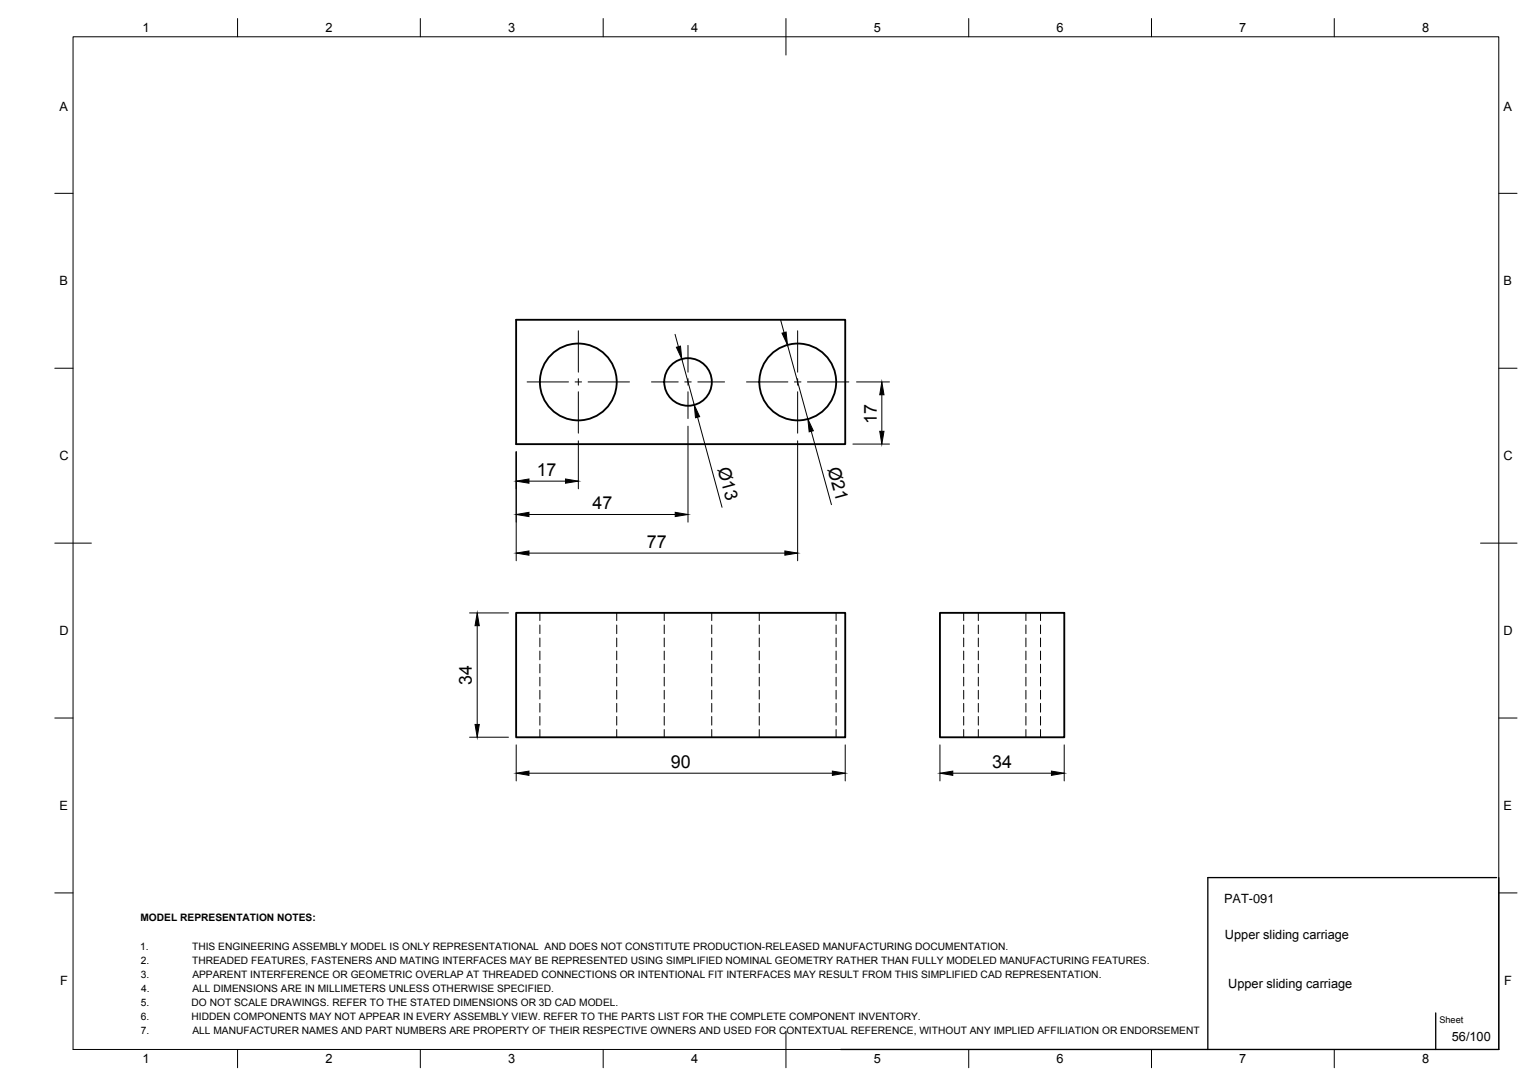
ISO-10303-21;
HEADER;
/* Generated by software containing ST-Developer
 * from STEP Tools, Inc. (www.steptools.com) 
 */

FILE_DESCRIPTION(
/* description */ ('PAT-091'),
/* implementation_level */ '2;1');

FILE_NAME(
/* name */ 'Upper sliding carriage.step',
/* time_stamp */ '2026-10-27T15:34:44-07:00',
/* author */ (''),
/* organization */ (''),
/* preprocessor_version */ 'ST-DEVELOPER v20.2',
/* originating_system */ 'Autodesk Translation Framework v15.17.0.0',
/* authorisation */ '');

FILE_SCHEMA (('AUTOMOTIVE_DESIGN { 1 0 10303 214 3 1 1 }'));
ENDSEC;

DATA;
#10=MECHANICAL_DESIGN_GEOMETRIC_PRESENTATION_REPRESENTATION('',(#1013),#25100);
#793=SHAPE_REPRESENTATION_RELATIONSHIP('SRR','None',#25557,#903);
#903=ADVANCED_BREP_SHAPE_REPRESENTATION('',(#1135),#25027);
#1013=STYLED_ITEM('',(#26177),#1135);
#1135=MANIFOLD_SOLID_BREP('Body1',#13292);
#1432=FACE_BOUND('',#3439,.T.);
#1433=FACE_BOUND('',#3440,.T.);
#1434=FACE_BOUND('',#3441,.T.);
#1435=FACE_BOUND('',#3444,.T.);
#1436=FACE_BOUND('',#3445,.T.);
#1437=FACE_BOUND('',#3446,.T.);
#1823=PLANE('',#15279);
#1824=PLANE('',#15280);
#1825=PLANE('',#15281);
#1826=PLANE('',#15282);
#1827=PLANE('',#15283);
#1828=PLANE('',#15284);
#2399=FACE_OUTER_BOUND('',#3434,.T.);
#2400=FACE_OUTER_BOUND('',#3435,.T.);
#2401=FACE_OUTER_BOUND('',#3436,.T.);
#2402=FACE_OUTER_BOUND('',#3437,.T.);
#2403=FACE_OUTER_BOUND('',#3438,.T.);
#2404=FACE_OUTER_BOUND('',#3442,.T.);
#2405=FACE_OUTER_BOUND('',#3443,.T.);
#2406=FACE_OUTER_BOUND('',#3447,.T.);
#2407=FACE_OUTER_BOUND('',#3448,.T.);
#3434=EDGE_LOOP('',(#10344,#10345,#10346,#10347));
#3435=EDGE_LOOP('',(#10348,#10349,#10350,#10351));
#3436=EDGE_LOOP('',(#10352,#10353,#10354,#10355));
#3437=EDGE_LOOP('',(#10356,#10357,#10358,#10359));
#3438=EDGE_LOOP('',(#10360,#10361,#10362,#10363));
#3439=EDGE_LOOP('',(#10364));
#3440=EDGE_LOOP('',(#10365));
#3441=EDGE_LOOP('',(#10366));
#3442=EDGE_LOOP('',(#10367,#10368,#10369,#10370));
#3443=EDGE_LOOP('',(#10371,#10372,#10373,#10374));
#3444=EDGE_LOOP('',(#10375));
#3445=EDGE_LOOP('',(#10376));
#3446=EDGE_LOOP('',(#10377));
#3447=EDGE_LOOP('',(#10378,#10379,#10380,#10381));
#3448=EDGE_LOOP('',(#10382,#10383,#10384,#10385));
#4507=LINE('',#22529,#5247);
#4508=LINE('',#22535,#5248);
#4509=LINE('',#22541,#5249);
#4510=LINE('',#22546,#5250);
#4511=LINE('',#22548,#5251);
#4512=LINE('',#22550,#5252);
#4513=LINE('',#22551,#5253);
#4514=LINE('',#22554,#5254);
#4515=LINE('',#22556,#5255);
#4516=LINE('',#22557,#5256);
#4517=LINE('',#22560,#5257);
#4518=LINE('',#22562,#5258);
#4519=LINE('',#22563,#5259);
#4520=LINE('',#22565,#5260);
#4521=LINE('',#22566,#5261);
#5247=VECTOR('',#18225,0.65);
#5248=VECTOR('',#18232,1.05);
#5249=VECTOR('',#18239,1.05);
#5250=VECTOR('',#18244,1.);
#5251=VECTOR('',#18245,1.);
#5252=VECTOR('',#18246,1.);
#5253=VECTOR('',#18247,1.);
#5254=VECTOR('',#18250,1.);
#5255=VECTOR('',#18251,1.);
#5256=VECTOR('',#18252,1.);
#5257=VECTOR('',#18255,1.);
#5258=VECTOR('',#18256,1.);
#5259=VECTOR('',#18257,1.);
#5260=VECTOR('',#18260,1.);
#5261=VECTOR('',#18261,1.);
#5905=CIRCLE('',#15271,0.65);
#5906=CIRCLE('',#15272,0.65);
#5907=CIRCLE('',#15274,1.05);
#5908=CIRCLE('',#15275,1.05);
#5909=CIRCLE('',#15277,1.05);
#5910=CIRCLE('',#15278,1.05);
#6838=VERTEX_POINT('',#22526);
#6839=VERTEX_POINT('',#22528);
#6840=VERTEX_POINT('',#22532);
#6841=VERTEX_POINT('',#22534);
#6842=VERTEX_POINT('',#22538);
#6843=VERTEX_POINT('',#22540);
#6844=VERTEX_POINT('',#22544);
#6845=VERTEX_POINT('',#22545);
#6846=VERTEX_POINT('',#22547);
#6847=VERTEX_POINT('',#22549);
#6848=VERTEX_POINT('',#22553);
#6849=VERTEX_POINT('',#22555);
#6850=VERTEX_POINT('',#22559);
#6851=VERTEX_POINT('',#22561);
#8107=EDGE_CURVE('',#6838,#6838,#5905,.T.);
#8108=EDGE_CURVE('',#6838,#6839,#4507,.T.);
#8109=EDGE_CURVE('',#6839,#6839,#5906,.T.);
#8110=EDGE_CURVE('',#6840,#6840,#5907,.T.);
#8111=EDGE_CURVE('',#6840,#6841,#4508,.T.);
#8112=EDGE_CURVE('',#6841,#6841,#5908,.T.);
#8113=EDGE_CURVE('',#6842,#6842,#5909,.T.);
#8114=EDGE_CURVE('',#6842,#6843,#4509,.T.);
#8115=EDGE_CURVE('',#6843,#6843,#5910,.T.);
#8116=EDGE_CURVE('',#6844,#6845,#4510,.T.);
#8117=EDGE_CURVE('',#6845,#6846,#4511,.T.);
#8118=EDGE_CURVE('',#6847,#6846,#4512,.T.);
#8119=EDGE_CURVE('',#6844,#6847,#4513,.T.);
#8120=EDGE_CURVE('',#6848,#6844,#4514,.T.);
#8121=EDGE_CURVE('',#6849,#6847,#4515,.T.);
#8122=EDGE_CURVE('',#6848,#6849,#4516,.T.);
#8123=EDGE_CURVE('',#6850,#6848,#4517,.T.);
#8124=EDGE_CURVE('',#6851,#6849,#4518,.T.);
#8125=EDGE_CURVE('',#6850,#6851,#4519,.T.);
#8126=EDGE_CURVE('',#6845,#6850,#4520,.T.);
#8127=EDGE_CURVE('',#6846,#6851,#4521,.T.);
#10344=ORIENTED_EDGE('',*,*,#8107,.F.);
#10345=ORIENTED_EDGE('',*,*,#8108,.T.);
#10346=ORIENTED_EDGE('',*,*,#8109,.F.);
#10347=ORIENTED_EDGE('',*,*,#8108,.F.);
#10348=ORIENTED_EDGE('',*,*,#8110,.F.);
#10349=ORIENTED_EDGE('',*,*,#8111,.T.);
#10350=ORIENTED_EDGE('',*,*,#8112,.F.);
#10351=ORIENTED_EDGE('',*,*,#8111,.F.);
#10352=ORIENTED_EDGE('',*,*,#8113,.F.);
#10353=ORIENTED_EDGE('',*,*,#8114,.T.);
#10354=ORIENTED_EDGE('',*,*,#8115,.F.);
#10355=ORIENTED_EDGE('',*,*,#8114,.F.);
#10356=ORIENTED_EDGE('',*,*,#8116,.T.);
#10357=ORIENTED_EDGE('',*,*,#8117,.T.);
#10358=ORIENTED_EDGE('',*,*,#8118,.F.);
#10359=ORIENTED_EDGE('',*,*,#8119,.F.);
#10360=ORIENTED_EDGE('',*,*,#8120,.T.);
#10361=ORIENTED_EDGE('',*,*,#8119,.T.);
#10362=ORIENTED_EDGE('',*,*,#8121,.F.);
#10363=ORIENTED_EDGE('',*,*,#8122,.F.);
#10364=ORIENTED_EDGE('',*,*,#8109,.T.);
#10365=ORIENTED_EDGE('',*,*,#8112,.T.);
#10366=ORIENTED_EDGE('',*,*,#8115,.T.);
#10367=ORIENTED_EDGE('',*,*,#8123,.T.);
#10368=ORIENTED_EDGE('',*,*,#8122,.T.);
#10369=ORIENTED_EDGE('',*,*,#8124,.F.);
#10370=ORIENTED_EDGE('',*,*,#8125,.F.);
#10371=ORIENTED_EDGE('',*,*,#8126,.T.);
#10372=ORIENTED_EDGE('',*,*,#8125,.T.);
#10373=ORIENTED_EDGE('',*,*,#8127,.F.);
#10374=ORIENTED_EDGE('',*,*,#8117,.F.);
#10375=ORIENTED_EDGE('',*,*,#8107,.T.);
#10376=ORIENTED_EDGE('',*,*,#8110,.T.);
#10377=ORIENTED_EDGE('',*,*,#8113,.T.);
#10378=ORIENTED_EDGE('',*,*,#8127,.T.);
#10379=ORIENTED_EDGE('',*,*,#8124,.T.);
#10380=ORIENTED_EDGE('',*,*,#8121,.T.);
#10381=ORIENTED_EDGE('',*,*,#8118,.T.);
#10382=ORIENTED_EDGE('',*,*,#8126,.F.);
#10383=ORIENTED_EDGE('',*,*,#8116,.F.);
#10384=ORIENTED_EDGE('',*,*,#8120,.F.);
#10385=ORIENTED_EDGE('',*,*,#8123,.F.);
#12220=CYLINDRICAL_SURFACE('',#15270,0.65);
#12221=CYLINDRICAL_SURFACE('',#15273,1.05);
#12222=CYLINDRICAL_SURFACE('',#15276,1.05);
#12766=ADVANCED_FACE('',(#2399),#12220,.F.);
#12767=ADVANCED_FACE('',(#2400),#12221,.F.);
#12768=ADVANCED_FACE('',(#2401),#12222,.F.);
#12769=ADVANCED_FACE('',(#2402),#1823,.T.);
#12770=ADVANCED_FACE('',(#2403,#1432,#1433,#1434),#1824,.T.);
#12771=ADVANCED_FACE('',(#2404),#1825,.T.);
#12772=ADVANCED_FACE('',(#2405,#1435,#1436,#1437),#1826,.T.);
#12773=ADVANCED_FACE('',(#2406),#1827,.T.);
#12774=ADVANCED_FACE('',(#2407),#1828,.F.);
#13292=CLOSED_SHELL('',(#12766,#12767,#12768,#12769,#12770,#12771,#12772,
#12773,#12774));
#15269=AXIS2_PLACEMENT_3D('',#22524,#18219,#18220);
#15270=AXIS2_PLACEMENT_3D('',#22525,#18221,#18222);
#15271=AXIS2_PLACEMENT_3D('',#22527,#18223,#18224);
#15272=AXIS2_PLACEMENT_3D('',#22530,#18226,#18227);
#15273=AXIS2_PLACEMENT_3D('',#22531,#18228,#18229);
#15274=AXIS2_PLACEMENT_3D('',#22533,#18230,#18231);
#15275=AXIS2_PLACEMENT_3D('',#22536,#18233,#18234);
#15276=AXIS2_PLACEMENT_3D('',#22537,#18235,#18236);
#15277=AXIS2_PLACEMENT_3D('',#22539,#18237,#18238);
#15278=AXIS2_PLACEMENT_3D('',#22542,#18240,#18241);
#15279=AXIS2_PLACEMENT_3D('',#22543,#18242,#18243);
#15280=AXIS2_PLACEMENT_3D('',#22552,#18248,#18249);
#15281=AXIS2_PLACEMENT_3D('',#22558,#18253,#18254);
#15282=AXIS2_PLACEMENT_3D('',#22564,#18258,#18259);
#15283=AXIS2_PLACEMENT_3D('',#22567,#18262,#18263);
#15284=AXIS2_PLACEMENT_3D('',#22568,#18264,#18265);
#18219=DIRECTION('axis',(0.,0.,1.));
#18220=DIRECTION('refdir',(1.,0.,0.));
#18221=DIRECTION('center_axis',(1.,0.,0.));
#18222=DIRECTION('ref_axis',(0.,0.,-1.));
#18223=DIRECTION('center_axis',(1.,0.,0.));
#18224=DIRECTION('ref_axis',(0.,0.,-1.));
#18225=DIRECTION('',(1.,0.,0.));
#18226=DIRECTION('center_axis',(-1.,0.,0.));
#18227=DIRECTION('ref_axis',(0.,0.,-1.));
#18228=DIRECTION('center_axis',(1.,0.,0.));
#18229=DIRECTION('ref_axis',(0.,0.,-1.));
#18230=DIRECTION('center_axis',(1.,0.,0.));
#18231=DIRECTION('ref_axis',(0.,0.,-1.));
#18232=DIRECTION('',(1.,0.,0.));
#18233=DIRECTION('center_axis',(-1.,0.,0.));
#18234=DIRECTION('ref_axis',(0.,0.,-1.));
#18235=DIRECTION('center_axis',(1.,0.,0.));
#18236=DIRECTION('ref_axis',(0.,0.,-1.));
#18237=DIRECTION('center_axis',(1.,0.,0.));
#18238=DIRECTION('ref_axis',(0.,0.,-1.));
#18239=DIRECTION('',(1.,0.,0.));
#18240=DIRECTION('center_axis',(-1.,0.,0.));
#18241=DIRECTION('ref_axis',(0.,0.,-1.));
#18242=DIRECTION('center_axis',(0.,1.,0.));
#18243=DIRECTION('ref_axis',(-1.,0.,0.));
#18244=DIRECTION('',(-1.,0.,0.));
#18245=DIRECTION('',(0.,0.,1.));
#18246=DIRECTION('',(-1.,0.,0.));
#18247=DIRECTION('',(0.,0.,1.));
#18248=DIRECTION('center_axis',(1.,0.,0.));
#18249=DIRECTION('ref_axis',(0.,1.,0.));
#18250=DIRECTION('',(0.,1.,0.));
#18251=DIRECTION('',(0.,1.,0.));
#18252=DIRECTION('',(0.,0.,1.));
#18253=DIRECTION('center_axis',(0.,-1.,0.));
#18254=DIRECTION('ref_axis',(1.,0.,0.));
#18255=DIRECTION('',(1.,0.,0.));
#18256=DIRECTION('',(1.,0.,0.));
#18257=DIRECTION('',(0.,0.,1.));
#18258=DIRECTION('center_axis',(-1.,0.,0.));
#18259=DIRECTION('ref_axis',(0.,-1.,0.));
#18260=DIRECTION('',(0.,-1.,0.));
#18261=DIRECTION('',(0.,-1.,0.));
#18262=DIRECTION('center_axis',(0.,0.,1.));
#18263=DIRECTION('ref_axis',(1.,0.,0.));
#18264=DIRECTION('center_axis',(0.,0.,1.));
#18265=DIRECTION('ref_axis',(1.,0.,0.));
#22524=CARTESIAN_POINT('',(0.,0.,0.));
#22525=CARTESIAN_POINT('Origin',(36.92983346,0.,16.));
#22526=CARTESIAN_POINT('',(37.0298334620742,-7.9602041944578E-17,16.65));
#22527=CARTESIAN_POINT('Origin',(37.0298334620742,0.,16.));
#22528=CARTESIAN_POINT('',(40.4298334620742,7.9602041944578E-17,16.65));
#22529=CARTESIAN_POINT('',(36.92983346,-7.9602041944578E-17,16.65));
#22530=CARTESIAN_POINT('Origin',(40.4298334620742,0.,16.));
#22531=CARTESIAN_POINT('Origin',(36.92983346,-3.,16.));
#22532=CARTESIAN_POINT('',(37.0298334620742,-3.,17.05));
#22533=CARTESIAN_POINT('Origin',(37.0298334620742,-3.,16.));
#22534=CARTESIAN_POINT('',(40.4298334620742,-3.,17.05));
#22535=CARTESIAN_POINT('',(36.92983346,-3.,17.05));
#22536=CARTESIAN_POINT('Origin',(40.4298334620742,-3.,16.));
#22537=CARTESIAN_POINT('Origin',(36.92983346,3.,16.));
#22538=CARTESIAN_POINT('',(37.0298334620742,3.,17.05));
#22539=CARTESIAN_POINT('Origin',(37.0298334620742,3.,16.));
#22540=CARTESIAN_POINT('',(40.4298334620742,3.,17.05));
#22541=CARTESIAN_POINT('',(36.92983346,3.,17.05));
#22542=CARTESIAN_POINT('Origin',(40.4298334620742,3.,16.));
#22543=CARTESIAN_POINT('Origin',(40.4298334620742,4.7,14.3));
#22544=CARTESIAN_POINT('',(40.4298334620742,4.7,14.3));
#22545=CARTESIAN_POINT('',(37.0298334620742,4.7,14.3));
#22546=CARTESIAN_POINT('',(40.4298334620742,4.7,14.3));
#22547=CARTESIAN_POINT('',(37.0298334620742,4.7,17.7));
#22548=CARTESIAN_POINT('',(37.0298334620742,4.7,14.3));
#22549=CARTESIAN_POINT('',(40.4298334620742,4.7,17.7));
#22550=CARTESIAN_POINT('',(40.4298334620742,4.7,17.7));
#22551=CARTESIAN_POINT('',(40.4298334620742,4.7,14.3));
#22552=CARTESIAN_POINT('Origin',(40.4298334620742,-4.3,14.3));
#22553=CARTESIAN_POINT('',(40.4298334620742,-4.3,14.3));
#22554=CARTESIAN_POINT('',(40.4298334620742,-4.3,14.3));
#22555=CARTESIAN_POINT('',(40.4298334620742,-4.3,17.7));
#22556=CARTESIAN_POINT('',(40.4298334620742,-4.3,17.7));
#22557=CARTESIAN_POINT('',(40.4298334620742,-4.3,14.3));
#22558=CARTESIAN_POINT('Origin',(37.0298334620742,-4.3,14.3));
#22559=CARTESIAN_POINT('',(37.0298334620742,-4.3,14.3));
#22560=CARTESIAN_POINT('',(37.0298334620742,-4.3,14.3));
#22561=CARTESIAN_POINT('',(37.0298334620742,-4.3,17.7));
#22562=CARTESIAN_POINT('',(37.0298334620742,-4.3,17.7));
#22563=CARTESIAN_POINT('',(37.0298334620742,-4.3,14.3));
#22564=CARTESIAN_POINT('Origin',(37.0298334620742,4.7,14.3));
#22565=CARTESIAN_POINT('',(37.0298334620742,4.7,14.3));
#22566=CARTESIAN_POINT('',(37.0298334620742,4.7,17.7));
#22567=CARTESIAN_POINT('Origin',(38.7298334620742,0.2,17.7));
#22568=CARTESIAN_POINT('Origin',(38.7298334620742,0.2,14.3));
#24906=UNCERTAINTY_MEASURE_WITH_UNIT(LENGTH_MEASURE(0.001),#25101,
'DISTANCE_ACCURACY_VALUE',
'Maximum model space distance between geometric entities at asserted c
onnectivities');
#24979=UNCERTAINTY_MEASURE_WITH_UNIT(LENGTH_MEASURE(0.001),#25101,
'DISTANCE_ACCURACY_VALUE',
'Maximum model space distance between geometric entities at asserted c
onnectivities');
#25027=(
GEOMETRIC_REPRESENTATION_CONTEXT(3)
GLOBAL_UNCERTAINTY_ASSIGNED_CONTEXT((#24906))
GLOBAL_UNIT_ASSIGNED_CONTEXT((#25101,#25103,#25104))
REPRESENTATION_CONTEXT('','3D')
);
#25100=(
GEOMETRIC_REPRESENTATION_CONTEXT(3)
GLOBAL_UNCERTAINTY_ASSIGNED_CONTEXT((#24979))
GLOBAL_UNIT_ASSIGNED_CONTEXT((#25101,#25103,#25104))
REPRESENTATION_CONTEXT('','3D')
);
#25101=(
LENGTH_UNIT()
NAMED_UNIT(*)
SI_UNIT(.CENTI.,.METRE.)
);
#25103=(
NAMED_UNIT(*)
PLANE_ANGLE_UNIT()
SI_UNIT($,.RADIAN.)
);
#25104=(
NAMED_UNIT(*)
SI_UNIT($,.STERADIAN.)
SOLID_ANGLE_UNIT()
);
#25152=SHAPE_DEFINITION_REPRESENTATION(#25272,#25557);
#25272=PRODUCT_DEFINITION_SHAPE('',$,#25678);
#25557=SHAPE_REPRESENTATION('',(#15269),#25027);
#25630=PRODUCT_DEFINITION_CONTEXT('part definition',#25992,'design');
#25678=PRODUCT_DEFINITION('Upper sliding carriage',
'Upper sliding carriage',#25798,#25630);
#25798=PRODUCT_DEFINITION_FORMATION('',$,#26041);
#25992=APPLICATION_CONTEXT(
'Core Data for Automotive Mechanical Design Process');
#25993=PRODUCT_CONTEXT('part definition',#25992,'mechanical');
#26041=PRODUCT('Upper sliding carriage','Upper sliding carriage',
'Upper sliding carriage',(#25993));
#26171=COLOUR_RGB('Light Blue',0.38,0.62,0.78);
#26172=FILL_AREA_STYLE_COLOUR('',#26171);
#26173=FILL_AREA_STYLE('',(#26172));
#26174=SURFACE_STYLE_FILL_AREA(#26173);
#26175=SURFACE_SIDE_STYLE('',(#26174));
#26176=SURFACE_STYLE_USAGE(.BOTH.,#26175);
#26177=PRESENTATION_STYLE_ASSIGNMENT((#26176));
ENDSEC;
END-ISO-10303-21;
